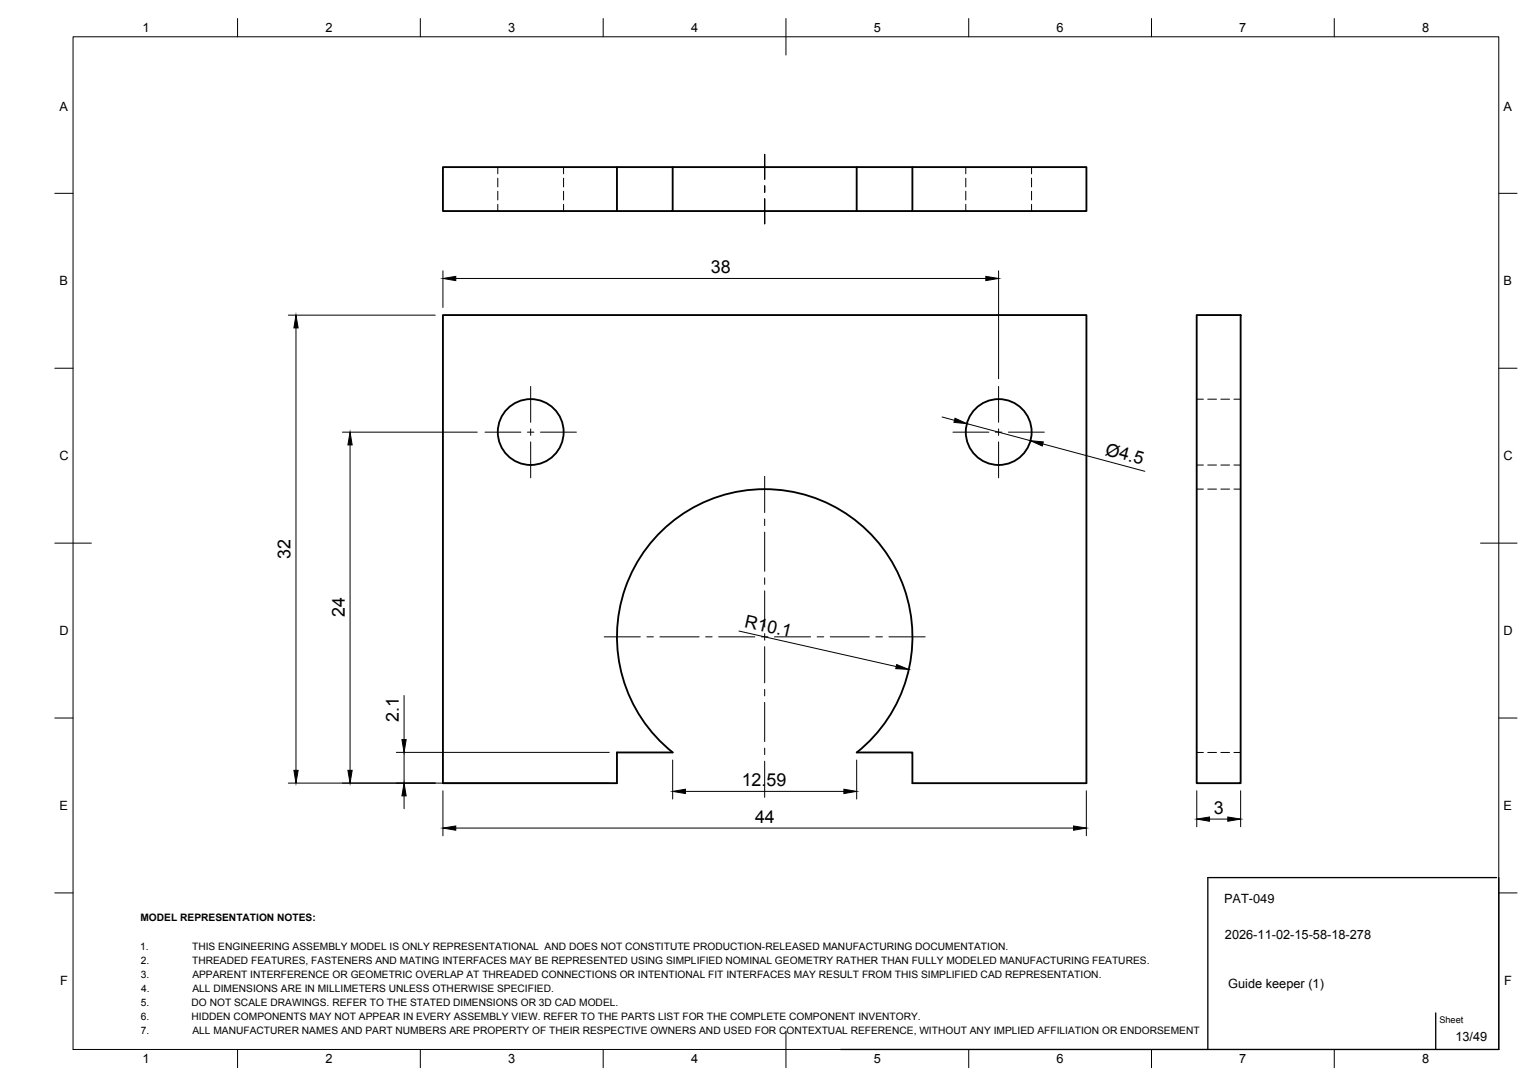
ISO-10303-21;
HEADER;
/* Generated by software containing ST-Developer
 * from STEP Tools, Inc. (www.steptools.com) 
 */

FILE_DESCRIPTION(
/* description */ ('Hand drill press frame (manual)'),
/* implementation_level */ '2;1');

FILE_NAME(
/* name */ 'Guide keeper (1).step',
/* time_stamp */ '2026-10-28T03:25:28-07:00',
/* author */ (''),
/* organization */ (''),
/* preprocessor_version */ 'ST-DEVELOPER v20.2',
/* originating_system */ 'Autodesk Translation Framework v15.17.0.0',
/* authorisation */ '');

FILE_SCHEMA (('AUTOMOTIVE_DESIGN { 1 0 10303 214 3 1 1 }'));
ENDSEC;

DATA;
#10=MECHANICAL_DESIGN_GEOMETRIC_PRESENTATION_REPRESENTATION('',(#627),#33299);
#537=SHAPE_REPRESENTATION_RELATIONSHIP('SRR','None',#33496,#582);
#582=ADVANCED_BREP_SHAPE_REPRESENTATION('',(#679),#33258);
#627=STYLED_ITEM('',(#33807),#679);
#679=MANIFOLD_SOLID_BREP('Body1',#12645);
#753=FACE_BOUND('',#2182,.T.);
#754=FACE_BOUND('',#2183,.T.);
#755=FACE_BOUND('',#2189,.T.);
#756=FACE_BOUND('',#2190,.T.);
#963=PLANE('',#13395);
#964=PLANE('',#13396);
#965=PLANE('',#13397);
#966=PLANE('',#13398);
#967=PLANE('',#13399);
#968=PLANE('',#13400);
#969=PLANE('',#13401);
#970=PLANE('',#13405);
#971=PLANE('',#13406);
#972=PLANE('',#13407);
#973=PLANE('',#13408);
#1451=FACE_OUTER_BOUND('',#2173,.T.);
#1452=FACE_OUTER_BOUND('',#2174,.T.);
#1453=FACE_OUTER_BOUND('',#2175,.T.);
#1454=FACE_OUTER_BOUND('',#2176,.T.);
#1455=FACE_OUTER_BOUND('',#2177,.T.);
#1456=FACE_OUTER_BOUND('',#2178,.T.);
#1457=FACE_OUTER_BOUND('',#2179,.T.);
#1458=FACE_OUTER_BOUND('',#2180,.T.);
#1459=FACE_OUTER_BOUND('',#2181,.T.);
#1460=FACE_OUTER_BOUND('',#2184,.T.);
#1461=FACE_OUTER_BOUND('',#2185,.T.);
#1462=FACE_OUTER_BOUND('',#2186,.T.);
#1463=FACE_OUTER_BOUND('',#2187,.T.);
#1464=FACE_OUTER_BOUND('',#2188,.T.);
#2173=EDGE_LOOP('',(#8955,#8956,#8957,#8958));
#2174=EDGE_LOOP('',(#8959,#8960,#8961,#8962));
#2175=EDGE_LOOP('',(#8963,#8964,#8965,#8966));
#2176=EDGE_LOOP('',(#8967,#8968,#8969,#8970));
#2177=EDGE_LOOP('',(#8971,#8972,#8973,#8974));
#2178=EDGE_LOOP('',(#8975,#8976,#8977,#8978));
#2179=EDGE_LOOP('',(#8979,#8980,#8981,#8982));
#2180=EDGE_LOOP('',(#8983,#8984,#8985,#8986));
#2181=EDGE_LOOP('',(#8987,#8988,#8989,#8990,#8991,#8992,#8993,#8994,#8995,
#8996));
#2182=EDGE_LOOP('',(#8997));
#2183=EDGE_LOOP('',(#8998));
#2184=EDGE_LOOP('',(#8999,#9000,#9001,#9002));
#2185=EDGE_LOOP('',(#9003,#9004,#9005,#9006));
#2186=EDGE_LOOP('',(#9007,#9008,#9009,#9010));
#2187=EDGE_LOOP('',(#9011,#9012,#9013,#9014));
#2188=EDGE_LOOP('',(#9015,#9016,#9017,#9018,#9019,#9020,#9021,#9022,#9023,
#9024));
#2189=EDGE_LOOP('',(#9025));
#2190=EDGE_LOOP('',(#9026));
#3063=LINE('',#18584,#4228);
#3064=LINE('',#18590,#4229);
#3065=LINE('',#18595,#4230);
#3066=LINE('',#18597,#4231);
#3067=LINE('',#18599,#4232);
#3068=LINE('',#18600,#4233);
#3069=LINE('',#18604,#4234);
#3070=LINE('',#18606,#4235);
#3071=LINE('',#18608,#4236);
#3072=LINE('',#18609,#4237);
#3073=LINE('',#18612,#4238);
#3074=LINE('',#18614,#4239);
#3075=LINE('',#18615,#4240);
#3076=LINE('',#18618,#4241);
#3077=LINE('',#18620,#4242);
#3078=LINE('',#18621,#4243);
#3079=LINE('',#18624,#4244);
#3080=LINE('',#18626,#4245);
#3081=LINE('',#18627,#4246);
#3082=LINE('',#18630,#4247);
#3083=LINE('',#18632,#4248);
#3084=LINE('',#18633,#4249);
#3085=LINE('',#18637,#4250);
#3086=LINE('',#18639,#4251);
#3087=LINE('',#18640,#4252);
#3088=LINE('',#18645,#4253);
#3089=LINE('',#18646,#4254);
#3090=LINE('',#18649,#4255);
#3091=LINE('',#18650,#4256);
#3092=LINE('',#18652,#4257);
#4228=VECTOR('',#14952,0.225);
#4229=VECTOR('',#14959,0.225);
#4230=VECTOR('',#14964,1.);
#4231=VECTOR('',#14965,1.);
#4232=VECTOR('',#14966,1.);
#4233=VECTOR('',#14967,1.);
#4234=VECTOR('',#14970,1.);
#4235=VECTOR('',#14971,1.);
#4236=VECTOR('',#14972,1.);
#4237=VECTOR('',#14973,1.);
#4238=VECTOR('',#14976,1.);
#4239=VECTOR('',#14977,1.);
#4240=VECTOR('',#14978,1.);
#4241=VECTOR('',#14981,1.);
#4242=VECTOR('',#14982,1.);
#4243=VECTOR('',#14983,1.);
#4244=VECTOR('',#14986,1.);
#4245=VECTOR('',#14987,1.);
#4246=VECTOR('',#14988,1.);
#4247=VECTOR('',#14991,1.);
#4248=VECTOR('',#14992,1.);
#4249=VECTOR('',#14993,1.);
#4250=VECTOR('',#14998,1.);
#4251=VECTOR('',#14999,1.);
#4252=VECTOR('',#15000,1.);
#4253=VECTOR('',#15007,1.);
#4254=VECTOR('',#15008,1.);
#4255=VECTOR('',#15011,1.);
#4256=VECTOR('',#15012,1.);
#4257=VECTOR('',#15015,1.);
#5292=CIRCLE('',#13390,0.225);
#5293=CIRCLE('',#13391,0.225);
#5294=CIRCLE('',#13393,0.225);
#5295=CIRCLE('',#13394,0.225);
#5296=CIRCLE('',#13402,1.01);
#5297=CIRCLE('',#13404,1.01);
#5791=VERTEX_POINT('',#18581);
#5792=VERTEX_POINT('',#18583);
#5793=VERTEX_POINT('',#18587);
#5794=VERTEX_POINT('',#18589);
#5795=VERTEX_POINT('',#18593);
#5796=VERTEX_POINT('',#18594);
#5797=VERTEX_POINT('',#18596);
#5798=VERTEX_POINT('',#18598);
#5799=VERTEX_POINT('',#18602);
#5800=VERTEX_POINT('',#18603);
#5801=VERTEX_POINT('',#18605);
#5802=VERTEX_POINT('',#18607);
#5803=VERTEX_POINT('',#18611);
#5804=VERTEX_POINT('',#18613);
#5805=VERTEX_POINT('',#18617);
#5806=VERTEX_POINT('',#18619);
#5807=VERTEX_POINT('',#18623);
#5808=VERTEX_POINT('',#18625);
#5809=VERTEX_POINT('',#18629);
#5810=VERTEX_POINT('',#18631);
#5811=VERTEX_POINT('',#18636);
#5812=VERTEX_POINT('',#18638);
#5813=VERTEX_POINT('',#18644);
#5814=VERTEX_POINT('',#18648);
#7006=EDGE_CURVE('',#5791,#5791,#5292,.T.);
#7007=EDGE_CURVE('',#5791,#5792,#3063,.T.);
#7008=EDGE_CURVE('',#5792,#5792,#5293,.T.);
#7009=EDGE_CURVE('',#5793,#5793,#5294,.T.);
#7010=EDGE_CURVE('',#5793,#5794,#3064,.T.);
#7011=EDGE_CURVE('',#5794,#5794,#5295,.T.);
#7012=EDGE_CURVE('',#5795,#5796,#3065,.T.);
#7013=EDGE_CURVE('',#5795,#5797,#3066,.T.);
#7014=EDGE_CURVE('',#5798,#5797,#3067,.T.);
#7015=EDGE_CURVE('',#5796,#5798,#3068,.T.);
#7016=EDGE_CURVE('',#5799,#5800,#3069,.T.);
#7017=EDGE_CURVE('',#5801,#5799,#3070,.T.);
#7018=EDGE_CURVE('',#5802,#5801,#3071,.T.);
#7019=EDGE_CURVE('',#5800,#5802,#3072,.T.);
#7020=EDGE_CURVE('',#5803,#5799,#3073,.T.);
#7021=EDGE_CURVE('',#5804,#5803,#3074,.T.);
#7022=EDGE_CURVE('',#5801,#5804,#3075,.T.);
#7023=EDGE_CURVE('',#5805,#5795,#3076,.T.);
#7024=EDGE_CURVE('',#5806,#5805,#3077,.T.);
#7025=EDGE_CURVE('',#5797,#5806,#3078,.T.);
#7026=EDGE_CURVE('',#5807,#5798,#3079,.T.);
#7027=EDGE_CURVE('',#5808,#5807,#3080,.T.);
#7028=EDGE_CURVE('',#5808,#5796,#3081,.T.);
#7029=EDGE_CURVE('',#5802,#5809,#3082,.T.);
#7030=EDGE_CURVE('',#5809,#5810,#3083,.T.);
#7031=EDGE_CURVE('',#5800,#5810,#3084,.T.);
#7032=EDGE_CURVE('',#5806,#5803,#5296,.T.);
#7033=EDGE_CURVE('',#5810,#5811,#3085,.T.);
#7034=EDGE_CURVE('',#5811,#5812,#3086,.T.);
#7035=EDGE_CURVE('',#5812,#5807,#3087,.T.);
#7036=EDGE_CURVE('',#5804,#5805,#5297,.T.);
#7037=EDGE_CURVE('',#5813,#5808,#3088,.T.);
#7038=EDGE_CURVE('',#5813,#5812,#3089,.T.);
#7039=EDGE_CURVE('',#5814,#5813,#3090,.T.);
#7040=EDGE_CURVE('',#5814,#5811,#3091,.T.);
#7041=EDGE_CURVE('',#5809,#5814,#3092,.T.);
#8955=ORIENTED_EDGE('',*,*,#7006,.F.);
#8956=ORIENTED_EDGE('',*,*,#7007,.T.);
#8957=ORIENTED_EDGE('',*,*,#7008,.F.);
#8958=ORIENTED_EDGE('',*,*,#7007,.F.);
#8959=ORIENTED_EDGE('',*,*,#7009,.F.);
#8960=ORIENTED_EDGE('',*,*,#7010,.T.);
#8961=ORIENTED_EDGE('',*,*,#7011,.F.);
#8962=ORIENTED_EDGE('',*,*,#7010,.F.);
#8963=ORIENTED_EDGE('',*,*,#7012,.F.);
#8964=ORIENTED_EDGE('',*,*,#7013,.T.);
#8965=ORIENTED_EDGE('',*,*,#7014,.F.);
#8966=ORIENTED_EDGE('',*,*,#7015,.F.);
#8967=ORIENTED_EDGE('',*,*,#7016,.F.);
#8968=ORIENTED_EDGE('',*,*,#7017,.F.);
#8969=ORIENTED_EDGE('',*,*,#7018,.F.);
#8970=ORIENTED_EDGE('',*,*,#7019,.F.);
#8971=ORIENTED_EDGE('',*,*,#7020,.F.);
#8972=ORIENTED_EDGE('',*,*,#7021,.F.);
#8973=ORIENTED_EDGE('',*,*,#7022,.F.);
#8974=ORIENTED_EDGE('',*,*,#7017,.T.);
#8975=ORIENTED_EDGE('',*,*,#7023,.F.);
#8976=ORIENTED_EDGE('',*,*,#7024,.F.);
#8977=ORIENTED_EDGE('',*,*,#7025,.F.);
#8978=ORIENTED_EDGE('',*,*,#7013,.F.);
#8979=ORIENTED_EDGE('',*,*,#7015,.T.);
#8980=ORIENTED_EDGE('',*,*,#7026,.F.);
#8981=ORIENTED_EDGE('',*,*,#7027,.F.);
#8982=ORIENTED_EDGE('',*,*,#7028,.T.);
#8983=ORIENTED_EDGE('',*,*,#7019,.T.);
#8984=ORIENTED_EDGE('',*,*,#7029,.T.);
#8985=ORIENTED_EDGE('',*,*,#7030,.T.);
#8986=ORIENTED_EDGE('',*,*,#7031,.F.);
#8987=ORIENTED_EDGE('',*,*,#7014,.T.);
#8988=ORIENTED_EDGE('',*,*,#7025,.T.);
#8989=ORIENTED_EDGE('',*,*,#7032,.T.);
#8990=ORIENTED_EDGE('',*,*,#7020,.T.);
#8991=ORIENTED_EDGE('',*,*,#7016,.T.);
#8992=ORIENTED_EDGE('',*,*,#7031,.T.);
#8993=ORIENTED_EDGE('',*,*,#7033,.T.);
#8994=ORIENTED_EDGE('',*,*,#7034,.T.);
#8995=ORIENTED_EDGE('',*,*,#7035,.T.);
#8996=ORIENTED_EDGE('',*,*,#7026,.T.);
#8997=ORIENTED_EDGE('',*,*,#7008,.T.);
#8998=ORIENTED_EDGE('',*,*,#7011,.T.);
#8999=ORIENTED_EDGE('',*,*,#7024,.T.);
#9000=ORIENTED_EDGE('',*,*,#7036,.F.);
#9001=ORIENTED_EDGE('',*,*,#7021,.T.);
#9002=ORIENTED_EDGE('',*,*,#7032,.F.);
#9003=ORIENTED_EDGE('',*,*,#7037,.T.);
#9004=ORIENTED_EDGE('',*,*,#7027,.T.);
#9005=ORIENTED_EDGE('',*,*,#7035,.F.);
#9006=ORIENTED_EDGE('',*,*,#7038,.F.);
#9007=ORIENTED_EDGE('',*,*,#7039,.T.);
#9008=ORIENTED_EDGE('',*,*,#7038,.T.);
#9009=ORIENTED_EDGE('',*,*,#7034,.F.);
#9010=ORIENTED_EDGE('',*,*,#7040,.F.);
#9011=ORIENTED_EDGE('',*,*,#7041,.T.);
#9012=ORIENTED_EDGE('',*,*,#7040,.T.);
#9013=ORIENTED_EDGE('',*,*,#7033,.F.);
#9014=ORIENTED_EDGE('',*,*,#7030,.F.);
#9015=ORIENTED_EDGE('',*,*,#7012,.T.);
#9016=ORIENTED_EDGE('',*,*,#7028,.F.);
#9017=ORIENTED_EDGE('',*,*,#7037,.F.);
#9018=ORIENTED_EDGE('',*,*,#7039,.F.);
#9019=ORIENTED_EDGE('',*,*,#7041,.F.);
#9020=ORIENTED_EDGE('',*,*,#7029,.F.);
#9021=ORIENTED_EDGE('',*,*,#7018,.T.);
#9022=ORIENTED_EDGE('',*,*,#7022,.T.);
#9023=ORIENTED_EDGE('',*,*,#7036,.T.);
#9024=ORIENTED_EDGE('',*,*,#7023,.T.);
#9025=ORIENTED_EDGE('',*,*,#7006,.T.);
#9026=ORIENTED_EDGE('',*,*,#7009,.T.);
#11821=CYLINDRICAL_SURFACE('',#13389,0.225);
#11822=CYLINDRICAL_SURFACE('',#13392,0.225);
#11823=CYLINDRICAL_SURFACE('',#13403,1.01);
#12060=ADVANCED_FACE('',(#1451),#11821,.F.);
#12061=ADVANCED_FACE('',(#1452),#11822,.F.);
#12062=ADVANCED_FACE('',(#1453),#963,.F.);
#12063=ADVANCED_FACE('',(#1454),#964,.F.);
#12064=ADVANCED_FACE('',(#1455),#965,.F.);
#12065=ADVANCED_FACE('',(#1456),#966,.F.);
#12066=ADVANCED_FACE('',(#1457),#967,.T.);
#12067=ADVANCED_FACE('',(#1458),#968,.T.);
#12068=ADVANCED_FACE('',(#1459,#753,#754),#969,.T.);
#12069=ADVANCED_FACE('',(#1460),#11823,.F.);
#12070=ADVANCED_FACE('',(#1461),#970,.T.);
#12071=ADVANCED_FACE('',(#1462),#971,.T.);
#12072=ADVANCED_FACE('',(#1463),#972,.T.);
#12073=ADVANCED_FACE('',(#1464,#755,#756),#973,.F.);
#12645=CLOSED_SHELL('',(#12060,#12061,#12062,#12063,#12064,#12065,#12066,
#12067,#12068,#12069,#12070,#12071,#12072,#12073));
#13388=AXIS2_PLACEMENT_3D('',#18579,#14946,#14947);
#13389=AXIS2_PLACEMENT_3D('',#18580,#14948,#14949);
#13390=AXIS2_PLACEMENT_3D('',#18582,#14950,#14951);
#13391=AXIS2_PLACEMENT_3D('',#18585,#14953,#14954);
#13392=AXIS2_PLACEMENT_3D('',#18586,#14955,#14956);
#13393=AXIS2_PLACEMENT_3D('',#18588,#14957,#14958);
#13394=AXIS2_PLACEMENT_3D('',#18591,#14960,#14961);
#13395=AXIS2_PLACEMENT_3D('',#18592,#14962,#14963);
#13396=AXIS2_PLACEMENT_3D('',#18601,#14968,#14969);
#13397=AXIS2_PLACEMENT_3D('',#18610,#14974,#14975);
#13398=AXIS2_PLACEMENT_3D('',#18616,#14979,#14980);
#13399=AXIS2_PLACEMENT_3D('',#18622,#14984,#14985);
#13400=AXIS2_PLACEMENT_3D('',#18628,#14989,#14990);
#13401=AXIS2_PLACEMENT_3D('',#18634,#14994,#14995);
#13402=AXIS2_PLACEMENT_3D('',#18635,#14996,#14997);
#13403=AXIS2_PLACEMENT_3D('',#18641,#15001,#15002);
#13404=AXIS2_PLACEMENT_3D('',#18642,#15003,#15004);
#13405=AXIS2_PLACEMENT_3D('',#18643,#15005,#15006);
#13406=AXIS2_PLACEMENT_3D('',#18647,#15009,#15010);
#13407=AXIS2_PLACEMENT_3D('',#18651,#15013,#15014);
#13408=AXIS2_PLACEMENT_3D('',#18653,#15016,#15017);
#14946=DIRECTION('axis',(0.,0.,1.));
#14947=DIRECTION('refdir',(1.,0.,0.));
#14948=DIRECTION('center_axis',(0.,0.,1.));
#14949=DIRECTION('ref_axis',(1.,0.,0.));
#14950=DIRECTION('center_axis',(0.,0.,1.));
#14951=DIRECTION('ref_axis',(1.,0.,0.));
#14952=DIRECTION('',(0.,0.,1.));
#14953=DIRECTION('center_axis',(0.,0.,-1.));
#14954=DIRECTION('ref_axis',(1.,0.,0.));
#14955=DIRECTION('center_axis',(0.,0.,1.));
#14956=DIRECTION('ref_axis',(1.,0.,0.));
#14957=DIRECTION('center_axis',(0.,0.,1.));
#14958=DIRECTION('ref_axis',(1.,0.,0.));
#14959=DIRECTION('',(0.,0.,1.));
#14960=DIRECTION('center_axis',(0.,0.,-1.));
#14961=DIRECTION('ref_axis',(1.,0.,0.));
#14962=DIRECTION('center_axis',(0.,1.,0.));
#14963=DIRECTION('ref_axis',(-1.,0.,0.));
#14964=DIRECTION('',(-1.,0.,0.));
#14965=DIRECTION('',(0.,0.,1.));
#14966=DIRECTION('',(1.,0.,0.));
#14967=DIRECTION('',(0.,0.,1.));
#14968=DIRECTION('center_axis',(0.,-1.,0.));
#14969=DIRECTION('ref_axis',(1.,0.,0.));
#14970=DIRECTION('',(-1.,0.,0.));
#14971=DIRECTION('',(0.,0.,1.));
#14972=DIRECTION('',(1.,0.,0.));
#14973=DIRECTION('',(0.,0.,-1.));
#14974=DIRECTION('center_axis',(1.,0.,0.));
#14975=DIRECTION('ref_axis',(0.,1.,0.));
#14976=DIRECTION('',(0.,-1.,0.));
#14977=DIRECTION('',(0.,0.,1.));
#14978=DIRECTION('',(0.,1.,0.));
#14979=DIRECTION('center_axis',(1.,0.,0.));
#14980=DIRECTION('ref_axis',(0.,1.,0.));
#14981=DIRECTION('',(0.,1.,0.));
#14982=DIRECTION('',(0.,0.,-1.));
#14983=DIRECTION('',(0.,-1.,0.));
#14984=DIRECTION('center_axis',(-1.,0.,0.));
#14985=DIRECTION('ref_axis',(0.,-1.,0.));
#14986=DIRECTION('',(0.,-1.,0.));
#14987=DIRECTION('',(0.,0.,1.));
#14988=DIRECTION('',(0.,-1.,0.));
#14989=DIRECTION('center_axis',(-1.,0.,0.));
#14990=DIRECTION('ref_axis',(0.,-1.,0.));
#14991=DIRECTION('',(0.,-1.,0.));
#14992=DIRECTION('',(0.,0.,1.));
#14993=DIRECTION('',(0.,-1.,0.));
#14994=DIRECTION('center_axis',(0.,0.,1.));
#14995=DIRECTION('ref_axis',(1.,0.,0.));
#14996=DIRECTION('center_axis',(0.,0.,-1.));
#14997=DIRECTION('ref_axis',(1.,0.,0.));
#14998=DIRECTION('',(1.,0.,0.));
#14999=DIRECTION('',(0.,1.,0.));
#15000=DIRECTION('',(-1.,0.,0.));
#15001=DIRECTION('center_axis',(0.,0.,1.));
#15002=DIRECTION('ref_axis',(1.,0.,0.));
#15003=DIRECTION('center_axis',(0.,0.,1.));
#15004=DIRECTION('ref_axis',(1.,0.,0.));
#15005=DIRECTION('center_axis',(0.,1.,0.));
#15006=DIRECTION('ref_axis',(-1.,0.,0.));
#15007=DIRECTION('',(-1.,0.,0.));
#15008=DIRECTION('',(0.,0.,1.));
#15009=DIRECTION('center_axis',(1.,0.,0.));
#15010=DIRECTION('ref_axis',(0.,1.,0.));
#15011=DIRECTION('',(0.,1.,0.));
#15012=DIRECTION('',(0.,0.,1.));
#15013=DIRECTION('center_axis',(0.,-1.,0.));
#15014=DIRECTION('ref_axis',(1.,0.,0.));
#15015=DIRECTION('',(1.,0.,0.));
#15016=DIRECTION('center_axis',(0.,0.,1.));
#15017=DIRECTION('ref_axis',(1.,0.,0.));
#18579=CARTESIAN_POINT('',(0.,0.,0.));
#18580=CARTESIAN_POINT('Origin',(2.4,-1.6,25.2));
#18581=CARTESIAN_POINT('',(2.175,-1.6,25.3));
#18582=CARTESIAN_POINT('Origin',(2.4,-1.6,25.3));
#18583=CARTESIAN_POINT('',(2.175,-1.6,25.6));
#18584=CARTESIAN_POINT('',(2.175,-1.6,25.2));
#18585=CARTESIAN_POINT('Origin',(2.4,-1.6,25.6));
#18586=CARTESIAN_POINT('Origin',(2.4,1.6,25.2));
#18587=CARTESIAN_POINT('',(2.175,1.6,25.3));
#18588=CARTESIAN_POINT('Origin',(2.4,1.6,25.3));
#18589=CARTESIAN_POINT('',(2.175,1.6,25.6));
#18590=CARTESIAN_POINT('',(2.175,1.6,25.2));
#18591=CARTESIAN_POINT('Origin',(2.4,1.6,25.6));
#18592=CARTESIAN_POINT('Origin',(0.21,1.01,25.2));
#18593=CARTESIAN_POINT('',(0.21,1.01,25.3));
#18594=CARTESIAN_POINT('',(0.,1.01,25.3));
#18595=CARTESIAN_POINT('',(0.905,1.01,25.3));
#18596=CARTESIAN_POINT('',(0.21,1.01,25.6));
#18597=CARTESIAN_POINT('',(0.21,1.01,25.2));
#18598=CARTESIAN_POINT('',(0.,1.01,25.6));
#18599=CARTESIAN_POINT('',(0.905,1.01,25.6));
#18600=CARTESIAN_POINT('',(0.,1.01,25.25));
#18601=CARTESIAN_POINT('Origin',(-0.1,-1.01,25.2));
#18602=CARTESIAN_POINT('',(0.21,-1.01,25.6));
#18603=CARTESIAN_POINT('',(0.,-1.01,25.6));
#18604=CARTESIAN_POINT('',(0.75,-1.01,25.6));
#18605=CARTESIAN_POINT('',(0.21,-1.01,25.3));
#18606=CARTESIAN_POINT('',(0.21,-1.01,25.2));
#18607=CARTESIAN_POINT('',(0.,-1.01,25.3));
#18608=CARTESIAN_POINT('',(0.75,-1.01,25.3));
#18609=CARTESIAN_POINT('',(0.,-1.01,25.25));
#18610=CARTESIAN_POINT('Origin',(0.21,-1.01,25.2));
#18611=CARTESIAN_POINT('',(0.21,-0.629285308902091,25.6));
#18612=CARTESIAN_POINT('',(0.21,-0.505,25.6));
#18613=CARTESIAN_POINT('',(0.21,-0.629285308902091,25.3));
#18614=CARTESIAN_POINT('',(0.21,-0.629285308902091,25.2));
#18615=CARTESIAN_POINT('',(0.21,-0.505,25.3));
#18616=CARTESIAN_POINT('Origin',(0.21,-1.01,25.2));
#18617=CARTESIAN_POINT('',(0.21,0.629285308902091,25.3));
#18618=CARTESIAN_POINT('',(0.21,-0.505,25.3));
#18619=CARTESIAN_POINT('',(0.21,0.629285308902091,25.6));
#18620=CARTESIAN_POINT('',(0.21,0.629285308902091,25.2));
#18621=CARTESIAN_POINT('',(0.21,-0.505,25.6));
#18622=CARTESIAN_POINT('Origin',(0.,2.2,25.3));
#18623=CARTESIAN_POINT('',(0.,2.2,25.6));
#18624=CARTESIAN_POINT('',(0.,2.2,25.6));
#18625=CARTESIAN_POINT('',(0.,2.2,25.3));
#18626=CARTESIAN_POINT('',(0.,2.2,25.3));
#18627=CARTESIAN_POINT('',(0.,2.2,25.3));
#18628=CARTESIAN_POINT('Origin',(0.,2.2,25.3));
#18629=CARTESIAN_POINT('',(0.,-2.2,25.3));
#18630=CARTESIAN_POINT('',(0.,2.2,25.3));
#18631=CARTESIAN_POINT('',(0.,-2.2,25.6));
#18632=CARTESIAN_POINT('',(0.,-2.2,25.3));
#18633=CARTESIAN_POINT('',(0.,2.2,25.6));
#18634=CARTESIAN_POINT('Origin',(1.6,0.,25.6));
#18635=CARTESIAN_POINT('Origin',(1.,0.,25.6));
#18636=CARTESIAN_POINT('',(3.2,-2.2,25.6));
#18637=CARTESIAN_POINT('',(0.,-2.2,25.6));
#18638=CARTESIAN_POINT('',(3.2,2.2,25.6));
#18639=CARTESIAN_POINT('',(3.2,-2.2,25.6));
#18640=CARTESIAN_POINT('',(3.2,2.2,25.6));
#18641=CARTESIAN_POINT('Origin',(1.,0.,25.2));
#18642=CARTESIAN_POINT('Origin',(1.,0.,25.3));
#18643=CARTESIAN_POINT('Origin',(3.2,2.2,25.3));
#18644=CARTESIAN_POINT('',(3.2,2.2,25.3));
#18645=CARTESIAN_POINT('',(3.2,2.2,25.3));
#18646=CARTESIAN_POINT('',(3.2,2.2,25.3));
#18647=CARTESIAN_POINT('Origin',(3.2,-2.2,25.3));
#18648=CARTESIAN_POINT('',(3.2,-2.2,25.3));
#18649=CARTESIAN_POINT('',(3.2,-2.2,25.3));
#18650=CARTESIAN_POINT('',(3.2,-2.2,25.3));
#18651=CARTESIAN_POINT('Origin',(0.,-2.2,25.3));
#18652=CARTESIAN_POINT('',(0.,-2.2,25.3));
#18653=CARTESIAN_POINT('Origin',(1.6,0.,25.3));
#33206=UNCERTAINTY_MEASURE_WITH_UNIT(LENGTH_MEASURE(0.001),#33300,
'DISTANCE_ACCURACY_VALUE',
'Maximum model space distance between geometric entities at asserted c
onnectivities');
#33247=UNCERTAINTY_MEASURE_WITH_UNIT(LENGTH_MEASURE(0.001),#33300,
'DISTANCE_ACCURACY_VALUE',
'Maximum model space distance between geometric entities at asserted c
onnectivities');
#33258=(
GEOMETRIC_REPRESENTATION_CONTEXT(3)
GLOBAL_UNCERTAINTY_ASSIGNED_CONTEXT((#33206))
GLOBAL_UNIT_ASSIGNED_CONTEXT((#33300,#33302,#33303))
REPRESENTATION_CONTEXT('','3D')
);
#33299=(
GEOMETRIC_REPRESENTATION_CONTEXT(3)
GLOBAL_UNCERTAINTY_ASSIGNED_CONTEXT((#33247))
GLOBAL_UNIT_ASSIGNED_CONTEXT((#33300,#33302,#33303))
REPRESENTATION_CONTEXT('','3D')
);
#33300=(
LENGTH_UNIT()
NAMED_UNIT(*)
SI_UNIT(.CENTI.,.METRE.)
);
#33302=(
NAMED_UNIT(*)
PLANE_ANGLE_UNIT()
SI_UNIT($,.RADIAN.)
);
#33303=(
NAMED_UNIT(*)
SI_UNIT($,.STERADIAN.)
SOLID_ANGLE_UNIT()
);
#33314=SHAPE_DEFINITION_REPRESENTATION(#33365,#33496);
#33365=PRODUCT_DEFINITION_SHAPE('',$,#33548);
#33496=SHAPE_REPRESENTATION('',(#13388),#33258);
#33537=PRODUCT_DEFINITION_CONTEXT('part definition',#33692,'design');
#33548=PRODUCT_DEFINITION('Guide keeper (1)','Guide keeper (1)',#33599,#33537);
#33599=PRODUCT_DEFINITION_FORMATION('',$,#33704);
#33692=APPLICATION_CONTEXT(
'Core Data for Automotive Mechanical Design Process');
#33693=PRODUCT_CONTEXT('part definition',#33692,'mechanical');
#33704=PRODUCT('Guide keeper (1)','Guide keeper (1)','Guide keeper (1)',(#33693));
#33801=COLOUR_RGB('Sky Blue',0.24,0.69,0.87);
#33802=FILL_AREA_STYLE_COLOUR('',#33801);
#33803=FILL_AREA_STYLE('',(#33802));
#33804=SURFACE_STYLE_FILL_AREA(#33803);
#33805=SURFACE_SIDE_STYLE('',(#33804));
#33806=SURFACE_STYLE_USAGE(.BOTH.,#33805);
#33807=PRESENTATION_STYLE_ASSIGNMENT((#33806));
ENDSEC;
END-ISO-10303-21;
